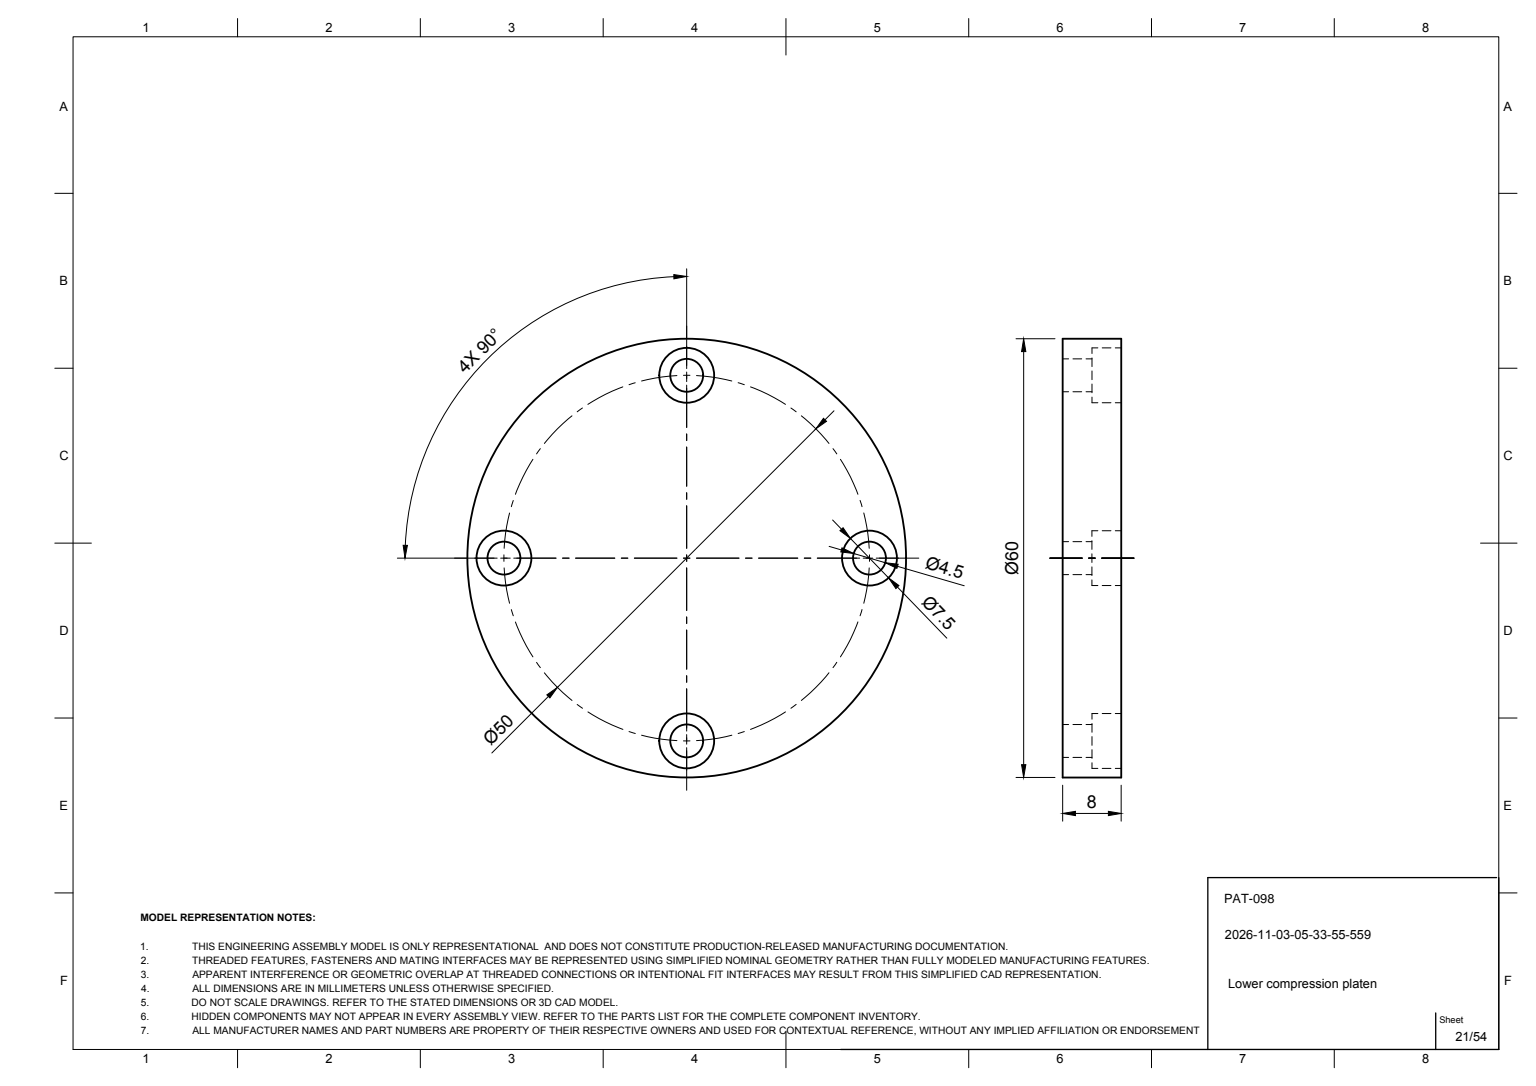
ISO-10303-21;
HEADER;
/* Generated by software containing ST-Developer
 * from STEP Tools, Inc. (www.steptools.com) 
 */

FILE_DESCRIPTION(
/* description */ ('Spring compression tester'),
/* implementation_level */ '2;1');

FILE_NAME(
/* name */ 'Lower compression platen.step',
/* time_stamp */ '2026-10-28T03:24:11-07:00',
/* author */ (''),
/* organization */ (''),
/* preprocessor_version */ 'ST-DEVELOPER v20.2',
/* originating_system */ 'Autodesk Translation Framework v15.17.0.0',
/* authorisation */ '');

FILE_SCHEMA (('AUTOMOTIVE_DESIGN { 1 0 10303 214 3 1 1 }'));
ENDSEC;

DATA;
#10=MECHANICAL_DESIGN_GEOMETRIC_PRESENTATION_REPRESENTATION('',(#1122),#43521);
#1002=SHAPE_REPRESENTATION_RELATIONSHIP('SRR','None',#43814,#1062);
#1062=ADVANCED_BREP_SHAPE_REPRESENTATION('',(#1197),#43474);
#1122=STYLED_ITEM('',(#44195),#1197);
#1197=MANIFOLD_SOLID_BREP('Body1',#18559);
#1398=FACE_BOUND('',#3604,.T.);
#1399=FACE_BOUND('',#3607,.T.);
#1400=FACE_BOUND('',#3610,.T.);
#1401=FACE_BOUND('',#3613,.T.);
#1402=FACE_BOUND('',#3620,.T.);
#1403=FACE_BOUND('',#3621,.T.);
#1404=FACE_BOUND('',#3622,.T.);
#1405=FACE_BOUND('',#3623,.T.);
#1406=FACE_BOUND('',#3625,.T.);
#1407=FACE_BOUND('',#3626,.T.);
#1408=FACE_BOUND('',#3627,.T.);
#1409=FACE_BOUND('',#3628,.T.);
#1722=PLANE('',#19752);
#1723=PLANE('',#19757);
#1724=PLANE('',#19762);
#1725=PLANE('',#19767);
#1726=PLANE('',#19780);
#1727=PLANE('',#19781);
#2404=FACE_OUTER_BOUND('',#3602,.T.);
#2405=FACE_OUTER_BOUND('',#3603,.T.);
#2406=FACE_OUTER_BOUND('',#3605,.T.);
#2407=FACE_OUTER_BOUND('',#3606,.T.);
#2408=FACE_OUTER_BOUND('',#3608,.T.);
#2409=FACE_OUTER_BOUND('',#3609,.T.);
#2410=FACE_OUTER_BOUND('',#3611,.T.);
#2411=FACE_OUTER_BOUND('',#3612,.T.);
#2412=FACE_OUTER_BOUND('',#3614,.T.);
#2413=FACE_OUTER_BOUND('',#3615,.T.);
#2414=FACE_OUTER_BOUND('',#3616,.T.);
#2415=FACE_OUTER_BOUND('',#3617,.T.);
#2416=FACE_OUTER_BOUND('',#3618,.T.);
#2417=FACE_OUTER_BOUND('',#3619,.T.);
#2418=FACE_OUTER_BOUND('',#3624,.T.);
#3602=EDGE_LOOP('',(#13231,#13232,#13233,#13234));
#3603=EDGE_LOOP('',(#13235));
#3604=EDGE_LOOP('',(#13236));
#3605=EDGE_LOOP('',(#13237,#13238,#13239,#13240));
#3606=EDGE_LOOP('',(#13241));
#3607=EDGE_LOOP('',(#13242));
#3608=EDGE_LOOP('',(#13243,#13244,#13245,#13246));
#3609=EDGE_LOOP('',(#13247));
#3610=EDGE_LOOP('',(#13248));
#3611=EDGE_LOOP('',(#13249,#13250,#13251,#13252));
#3612=EDGE_LOOP('',(#13253));
#3613=EDGE_LOOP('',(#13254));
#3614=EDGE_LOOP('',(#13255,#13256,#13257,#13258));
#3615=EDGE_LOOP('',(#13259,#13260,#13261,#13262));
#3616=EDGE_LOOP('',(#13263,#13264,#13265,#13266));
#3617=EDGE_LOOP('',(#13267,#13268,#13269,#13270));
#3618=EDGE_LOOP('',(#13271,#13272,#13273,#13274));
#3619=EDGE_LOOP('',(#13275));
#3620=EDGE_LOOP('',(#13276));
#3621=EDGE_LOOP('',(#13277));
#3622=EDGE_LOOP('',(#13278));
#3623=EDGE_LOOP('',(#13279));
#3624=EDGE_LOOP('',(#13280));
#3625=EDGE_LOOP('',(#13281));
#3626=EDGE_LOOP('',(#13282));
#3627=EDGE_LOOP('',(#13283));
#3628=EDGE_LOOP('',(#13284));
#4903=LINE('',#27556,#6335);
#4904=LINE('',#27565,#6336);
#4905=LINE('',#27574,#6337);
#4906=LINE('',#27583,#6338);
#4907=LINE('',#27591,#6339);
#4908=LINE('',#27595,#6340);
#4909=LINE('',#27599,#6341);
#4910=LINE('',#27603,#6342);
#4911=LINE('',#27608,#6343);
#6335=VECTOR('',#22427,0.375);
#6336=VECTOR('',#22438,0.375);
#6337=VECTOR('',#22449,0.375);
#6338=VECTOR('',#22460,0.375);
#6339=VECTOR('',#22471,0.225);
#6340=VECTOR('',#22476,0.225);
#6341=VECTOR('',#22481,0.225);
#6342=VECTOR('',#22486,0.225);
#6343=VECTOR('',#22491,3.);
#7680=CIRCLE('',#19750,0.375);
#7681=CIRCLE('',#19751,0.375);
#7682=CIRCLE('',#19753,0.225);
#7683=CIRCLE('',#19755,0.375);
#7684=CIRCLE('',#19756,0.375);
#7685=CIRCLE('',#19758,0.225);
#7686=CIRCLE('',#19760,0.375);
#7687=CIRCLE('',#19761,0.375);
#7688=CIRCLE('',#19763,0.225);
#7689=CIRCLE('',#19765,0.375);
#7690=CIRCLE('',#19766,0.375);
#7691=CIRCLE('',#19768,0.225);
#7692=CIRCLE('',#19770,0.225);
#7693=CIRCLE('',#19772,0.225);
#7694=CIRCLE('',#19774,0.225);
#7695=CIRCLE('',#19776,0.225);
#7696=CIRCLE('',#19778,3.);
#7697=CIRCLE('',#19779,3.);
#8474=VERTEX_POINT('',#27553);
#8475=VERTEX_POINT('',#27555);
#8476=VERTEX_POINT('',#27559);
#8477=VERTEX_POINT('',#27562);
#8478=VERTEX_POINT('',#27564);
#8479=VERTEX_POINT('',#27568);
#8480=VERTEX_POINT('',#27571);
#8481=VERTEX_POINT('',#27573);
#8482=VERTEX_POINT('',#27577);
#8483=VERTEX_POINT('',#27580);
#8484=VERTEX_POINT('',#27582);
#8485=VERTEX_POINT('',#27586);
#8486=VERTEX_POINT('',#27589);
#8487=VERTEX_POINT('',#27593);
#8488=VERTEX_POINT('',#27597);
#8489=VERTEX_POINT('',#27601);
#8490=VERTEX_POINT('',#27605);
#8491=VERTEX_POINT('',#27607);
#10280=EDGE_CURVE('',#8474,#8474,#7680,.T.);
#10281=EDGE_CURVE('',#8474,#8475,#4903,.T.);
#10282=EDGE_CURVE('',#8475,#8475,#7681,.T.);
#10283=EDGE_CURVE('',#8476,#8476,#7682,.T.);
#10284=EDGE_CURVE('',#8477,#8477,#7683,.T.);
#10285=EDGE_CURVE('',#8477,#8478,#4904,.T.);
#10286=EDGE_CURVE('',#8478,#8478,#7684,.T.);
#10287=EDGE_CURVE('',#8479,#8479,#7685,.T.);
#10288=EDGE_CURVE('',#8480,#8480,#7686,.T.);
#10289=EDGE_CURVE('',#8480,#8481,#4905,.T.);
#10290=EDGE_CURVE('',#8481,#8481,#7687,.T.);
#10291=EDGE_CURVE('',#8482,#8482,#7688,.T.);
#10292=EDGE_CURVE('',#8483,#8483,#7689,.T.);
#10293=EDGE_CURVE('',#8483,#8484,#4906,.T.);
#10294=EDGE_CURVE('',#8484,#8484,#7690,.T.);
#10295=EDGE_CURVE('',#8485,#8485,#7691,.T.);
#10296=EDGE_CURVE('',#8486,#8486,#7692,.T.);
#10297=EDGE_CURVE('',#8486,#8476,#4907,.T.);
#10298=EDGE_CURVE('',#8487,#8487,#7693,.T.);
#10299=EDGE_CURVE('',#8487,#8479,#4908,.T.);
#10300=EDGE_CURVE('',#8488,#8488,#7694,.T.);
#10301=EDGE_CURVE('',#8488,#8482,#4909,.T.);
#10302=EDGE_CURVE('',#8489,#8489,#7695,.T.);
#10303=EDGE_CURVE('',#8489,#8485,#4910,.T.);
#10304=EDGE_CURVE('',#8490,#8490,#7696,.T.);
#10305=EDGE_CURVE('',#8490,#8491,#4911,.T.);
#10306=EDGE_CURVE('',#8491,#8491,#7697,.T.);
#13231=ORIENTED_EDGE('',*,*,#10280,.F.);
#13232=ORIENTED_EDGE('',*,*,#10281,.T.);
#13233=ORIENTED_EDGE('',*,*,#10282,.F.);
#13234=ORIENTED_EDGE('',*,*,#10281,.F.);
#13235=ORIENTED_EDGE('',*,*,#10280,.T.);
#13236=ORIENTED_EDGE('',*,*,#10283,.F.);
#13237=ORIENTED_EDGE('',*,*,#10284,.F.);
#13238=ORIENTED_EDGE('',*,*,#10285,.T.);
#13239=ORIENTED_EDGE('',*,*,#10286,.F.);
#13240=ORIENTED_EDGE('',*,*,#10285,.F.);
#13241=ORIENTED_EDGE('',*,*,#10284,.T.);
#13242=ORIENTED_EDGE('',*,*,#10287,.F.);
#13243=ORIENTED_EDGE('',*,*,#10288,.F.);
#13244=ORIENTED_EDGE('',*,*,#10289,.T.);
#13245=ORIENTED_EDGE('',*,*,#10290,.F.);
#13246=ORIENTED_EDGE('',*,*,#10289,.F.);
#13247=ORIENTED_EDGE('',*,*,#10288,.T.);
#13248=ORIENTED_EDGE('',*,*,#10291,.F.);
#13249=ORIENTED_EDGE('',*,*,#10292,.F.);
#13250=ORIENTED_EDGE('',*,*,#10293,.T.);
#13251=ORIENTED_EDGE('',*,*,#10294,.F.);
#13252=ORIENTED_EDGE('',*,*,#10293,.F.);
#13253=ORIENTED_EDGE('',*,*,#10292,.T.);
#13254=ORIENTED_EDGE('',*,*,#10295,.F.);
#13255=ORIENTED_EDGE('',*,*,#10296,.F.);
#13256=ORIENTED_EDGE('',*,*,#10297,.T.);
#13257=ORIENTED_EDGE('',*,*,#10283,.T.);
#13258=ORIENTED_EDGE('',*,*,#10297,.F.);
#13259=ORIENTED_EDGE('',*,*,#10298,.F.);
#13260=ORIENTED_EDGE('',*,*,#10299,.T.);
#13261=ORIENTED_EDGE('',*,*,#10287,.T.);
#13262=ORIENTED_EDGE('',*,*,#10299,.F.);
#13263=ORIENTED_EDGE('',*,*,#10300,.F.);
#13264=ORIENTED_EDGE('',*,*,#10301,.T.);
#13265=ORIENTED_EDGE('',*,*,#10291,.T.);
#13266=ORIENTED_EDGE('',*,*,#10301,.F.);
#13267=ORIENTED_EDGE('',*,*,#10302,.F.);
#13268=ORIENTED_EDGE('',*,*,#10303,.T.);
#13269=ORIENTED_EDGE('',*,*,#10295,.T.);
#13270=ORIENTED_EDGE('',*,*,#10303,.F.);
#13271=ORIENTED_EDGE('',*,*,#10304,.F.);
#13272=ORIENTED_EDGE('',*,*,#10305,.T.);
#13273=ORIENTED_EDGE('',*,*,#10306,.T.);
#13274=ORIENTED_EDGE('',*,*,#10305,.F.);
#13275=ORIENTED_EDGE('',*,*,#10304,.T.);
#13276=ORIENTED_EDGE('',*,*,#10294,.T.);
#13277=ORIENTED_EDGE('',*,*,#10290,.T.);
#13278=ORIENTED_EDGE('',*,*,#10286,.T.);
#13279=ORIENTED_EDGE('',*,*,#10282,.T.);
#13280=ORIENTED_EDGE('',*,*,#10306,.F.);
#13281=ORIENTED_EDGE('',*,*,#10296,.T.);
#13282=ORIENTED_EDGE('',*,*,#10298,.T.);
#13283=ORIENTED_EDGE('',*,*,#10300,.T.);
#13284=ORIENTED_EDGE('',*,*,#10302,.T.);
#17206=CYLINDRICAL_SURFACE('',#19749,0.375);
#17207=CYLINDRICAL_SURFACE('',#19754,0.375);
#17208=CYLINDRICAL_SURFACE('',#19759,0.375);
#17209=CYLINDRICAL_SURFACE('',#19764,0.375);
#17210=CYLINDRICAL_SURFACE('',#19769,0.225);
#17211=CYLINDRICAL_SURFACE('',#19771,0.225);
#17212=CYLINDRICAL_SURFACE('',#19773,0.225);
#17213=CYLINDRICAL_SURFACE('',#19775,0.225);
#17214=CYLINDRICAL_SURFACE('',#19777,3.);
#17728=ADVANCED_FACE('',(#2404),#17206,.F.);
#17729=ADVANCED_FACE('',(#2405,#1398),#1722,.T.);
#17730=ADVANCED_FACE('',(#2406),#17207,.F.);
#17731=ADVANCED_FACE('',(#2407,#1399),#1723,.T.);
#17732=ADVANCED_FACE('',(#2408),#17208,.F.);
#17733=ADVANCED_FACE('',(#2409,#1400),#1724,.T.);
#17734=ADVANCED_FACE('',(#2410),#17209,.F.);
#17735=ADVANCED_FACE('',(#2411,#1401),#1725,.T.);
#17736=ADVANCED_FACE('',(#2412),#17210,.F.);
#17737=ADVANCED_FACE('',(#2413),#17211,.F.);
#17738=ADVANCED_FACE('',(#2414),#17212,.F.);
#17739=ADVANCED_FACE('',(#2415),#17213,.F.);
#17740=ADVANCED_FACE('',(#2416),#17214,.T.);
#17741=ADVANCED_FACE('',(#2417,#1402,#1403,#1404,#1405),#1726,.T.);
#17742=ADVANCED_FACE('',(#2418,#1406,#1407,#1408,#1409),#1727,.F.);
#18559=CLOSED_SHELL('',(#17728,#17729,#17730,#17731,#17732,#17733,#17734,
#17735,#17736,#17737,#17738,#17739,#17740,#17741,#17742));
#19748=AXIS2_PLACEMENT_3D('',#27551,#22421,#22422);
#19749=AXIS2_PLACEMENT_3D('',#27552,#22423,#22424);
#19750=AXIS2_PLACEMENT_3D('',#27554,#22425,#22426);
#19751=AXIS2_PLACEMENT_3D('',#27557,#22428,#22429);
#19752=AXIS2_PLACEMENT_3D('',#27558,#22430,#22431);
#19753=AXIS2_PLACEMENT_3D('',#27560,#22432,#22433);
#19754=AXIS2_PLACEMENT_3D('',#27561,#22434,#22435);
#19755=AXIS2_PLACEMENT_3D('',#27563,#22436,#22437);
#19756=AXIS2_PLACEMENT_3D('',#27566,#22439,#22440);
#19757=AXIS2_PLACEMENT_3D('',#27567,#22441,#22442);
#19758=AXIS2_PLACEMENT_3D('',#27569,#22443,#22444);
#19759=AXIS2_PLACEMENT_3D('',#27570,#22445,#22446);
#19760=AXIS2_PLACEMENT_3D('',#27572,#22447,#22448);
#19761=AXIS2_PLACEMENT_3D('',#27575,#22450,#22451);
#19762=AXIS2_PLACEMENT_3D('',#27576,#22452,#22453);
#19763=AXIS2_PLACEMENT_3D('',#27578,#22454,#22455);
#19764=AXIS2_PLACEMENT_3D('',#27579,#22456,#22457);
#19765=AXIS2_PLACEMENT_3D('',#27581,#22458,#22459);
#19766=AXIS2_PLACEMENT_3D('',#27584,#22461,#22462);
#19767=AXIS2_PLACEMENT_3D('',#27585,#22463,#22464);
#19768=AXIS2_PLACEMENT_3D('',#27587,#22465,#22466);
#19769=AXIS2_PLACEMENT_3D('',#27588,#22467,#22468);
#19770=AXIS2_PLACEMENT_3D('',#27590,#22469,#22470);
#19771=AXIS2_PLACEMENT_3D('',#27592,#22472,#22473);
#19772=AXIS2_PLACEMENT_3D('',#27594,#22474,#22475);
#19773=AXIS2_PLACEMENT_3D('',#27596,#22477,#22478);
#19774=AXIS2_PLACEMENT_3D('',#27598,#22479,#22480);
#19775=AXIS2_PLACEMENT_3D('',#27600,#22482,#22483);
#19776=AXIS2_PLACEMENT_3D('',#27602,#22484,#22485);
#19777=AXIS2_PLACEMENT_3D('',#27604,#22487,#22488);
#19778=AXIS2_PLACEMENT_3D('',#27606,#22489,#22490);
#19779=AXIS2_PLACEMENT_3D('',#27609,#22492,#22493);
#19780=AXIS2_PLACEMENT_3D('',#27610,#22494,#22495);
#19781=AXIS2_PLACEMENT_3D('',#27611,#22496,#22497);
#22421=DIRECTION('axis',(0.,0.,1.));
#22422=DIRECTION('refdir',(1.,0.,0.));
#22423=DIRECTION('center_axis',(0.,0.,1.));
#22424=DIRECTION('ref_axis',(1.,0.,0.));
#22425=DIRECTION('center_axis',(0.,0.,1.));
#22426=DIRECTION('ref_axis',(1.,0.,0.));
#22427=DIRECTION('',(0.,0.,1.));
#22428=DIRECTION('center_axis',(0.,0.,-1.));
#22429=DIRECTION('ref_axis',(1.,0.,0.));
#22430=DIRECTION('center_axis',(0.,0.,1.));
#22431=DIRECTION('ref_axis',(1.,0.,0.));
#22432=DIRECTION('center_axis',(0.,0.,1.));
#22433=DIRECTION('ref_axis',(1.,0.,0.));
#22434=DIRECTION('center_axis',(0.,0.,1.));
#22435=DIRECTION('ref_axis',(1.,0.,0.));
#22436=DIRECTION('center_axis',(0.,0.,1.));
#22437=DIRECTION('ref_axis',(1.,0.,0.));
#22438=DIRECTION('',(0.,0.,1.));
#22439=DIRECTION('center_axis',(0.,0.,-1.));
#22440=DIRECTION('ref_axis',(1.,0.,0.));
#22441=DIRECTION('center_axis',(0.,0.,1.));
#22442=DIRECTION('ref_axis',(1.,0.,0.));
#22443=DIRECTION('center_axis',(0.,0.,1.));
#22444=DIRECTION('ref_axis',(1.,0.,0.));
#22445=DIRECTION('center_axis',(0.,0.,1.));
#22446=DIRECTION('ref_axis',(1.,0.,0.));
#22447=DIRECTION('center_axis',(0.,0.,1.));
#22448=DIRECTION('ref_axis',(1.,0.,0.));
#22449=DIRECTION('',(0.,0.,1.));
#22450=DIRECTION('center_axis',(0.,0.,-1.));
#22451=DIRECTION('ref_axis',(1.,0.,0.));
#22452=DIRECTION('center_axis',(0.,0.,1.));
#22453=DIRECTION('ref_axis',(1.,0.,0.));
#22454=DIRECTION('center_axis',(0.,0.,1.));
#22455=DIRECTION('ref_axis',(1.,0.,0.));
#22456=DIRECTION('center_axis',(0.,0.,1.));
#22457=DIRECTION('ref_axis',(1.,0.,0.));
#22458=DIRECTION('center_axis',(0.,0.,1.));
#22459=DIRECTION('ref_axis',(1.,0.,0.));
#22460=DIRECTION('',(0.,0.,1.));
#22461=DIRECTION('center_axis',(0.,0.,-1.));
#22462=DIRECTION('ref_axis',(1.,0.,0.));
#22463=DIRECTION('center_axis',(0.,0.,1.));
#22464=DIRECTION('ref_axis',(1.,0.,0.));
#22465=DIRECTION('center_axis',(0.,0.,1.));
#22466=DIRECTION('ref_axis',(1.,0.,0.));
#22467=DIRECTION('center_axis',(0.,0.,1.));
#22468=DIRECTION('ref_axis',(1.,0.,0.));
#22469=DIRECTION('center_axis',(0.,0.,1.));
#22470=DIRECTION('ref_axis',(1.,0.,0.));
#22471=DIRECTION('',(0.,0.,1.));
#22472=DIRECTION('center_axis',(0.,0.,1.));
#22473=DIRECTION('ref_axis',(1.,0.,0.));
#22474=DIRECTION('center_axis',(0.,0.,1.));
#22475=DIRECTION('ref_axis',(1.,0.,0.));
#22476=DIRECTION('',(0.,0.,1.));
#22477=DIRECTION('center_axis',(0.,0.,1.));
#22478=DIRECTION('ref_axis',(1.,0.,0.));
#22479=DIRECTION('center_axis',(0.,0.,1.));
#22480=DIRECTION('ref_axis',(1.,0.,0.));
#22481=DIRECTION('',(0.,0.,1.));
#22482=DIRECTION('center_axis',(0.,0.,1.));
#22483=DIRECTION('ref_axis',(1.,0.,0.));
#22484=DIRECTION('center_axis',(0.,0.,1.));
#22485=DIRECTION('ref_axis',(1.,0.,0.));
#22486=DIRECTION('',(0.,0.,1.));
#22487=DIRECTION('center_axis',(0.,0.,1.));
#22488=DIRECTION('ref_axis',(1.,0.,0.));
#22489=DIRECTION('center_axis',(0.,0.,1.));
#22490=DIRECTION('ref_axis',(1.,0.,0.));
#22491=DIRECTION('',(0.,0.,-1.));
#22492=DIRECTION('center_axis',(0.,0.,1.));
#22493=DIRECTION('ref_axis',(1.,0.,0.));
#22494=DIRECTION('center_axis',(0.,0.,1.));
#22495=DIRECTION('ref_axis',(1.,0.,0.));
#22496=DIRECTION('center_axis',(0.,0.,1.));
#22497=DIRECTION('ref_axis',(1.,0.,0.));
#27551=CARTESIAN_POINT('',(0.,0.,0.));
#27552=CARTESIAN_POINT('Origin',(-2.5,-1.5,0.4));
#27553=CARTESIAN_POINT('',(-2.875,-1.5,0.4));
#27554=CARTESIAN_POINT('Origin',(-2.5,-1.5,0.4));
#27555=CARTESIAN_POINT('',(-2.875,-1.5,0.8));
#27556=CARTESIAN_POINT('',(-2.875,-1.5,0.4));
#27557=CARTESIAN_POINT('Origin',(-2.5,-1.5,0.8));
#27558=CARTESIAN_POINT('Origin',(-2.5,-1.5,0.4));
#27559=CARTESIAN_POINT('',(-2.725,-1.5,0.4));
#27560=CARTESIAN_POINT('Origin',(-2.5,-1.5,0.4));
#27561=CARTESIAN_POINT('Origin',(1.53080849893419E-16,1.,0.4));
#27562=CARTESIAN_POINT('',(-0.375,1.,0.4));
#27563=CARTESIAN_POINT('Origin',(1.53080849893419E-16,1.,0.4));
#27564=CARTESIAN_POINT('',(-0.375,1.,0.8));
#27565=CARTESIAN_POINT('',(-0.375,1.,0.4));
#27566=CARTESIAN_POINT('Origin',(1.53080849893419E-16,1.,0.8));
#27567=CARTESIAN_POINT('Origin',(1.66533453693773E-16,1.,0.4));
#27568=CARTESIAN_POINT('',(-0.225,1.,0.4));
#27569=CARTESIAN_POINT('Origin',(1.53080849893419E-16,1.,0.4));
#27570=CARTESIAN_POINT('Origin',(2.5,-1.5,0.4));
#27571=CARTESIAN_POINT('',(2.125,-1.5,0.4));
#27572=CARTESIAN_POINT('Origin',(2.5,-1.5,0.4));
#27573=CARTESIAN_POINT('',(2.125,-1.5,0.8));
#27574=CARTESIAN_POINT('',(2.125,-1.5,0.4));
#27575=CARTESIAN_POINT('Origin',(2.5,-1.5,0.8));
#27576=CARTESIAN_POINT('Origin',(2.5,-1.5,0.4));
#27577=CARTESIAN_POINT('',(2.275,-1.5,0.4));
#27578=CARTESIAN_POINT('Origin',(2.5,-1.5,0.4));
#27579=CARTESIAN_POINT('Origin',(-4.59242549680257E-16,-4.,0.4));
#27580=CARTESIAN_POINT('',(-0.375,-4.,0.4));
#27581=CARTESIAN_POINT('Origin',(-4.59242549680257E-16,-4.,0.4));
#27582=CARTESIAN_POINT('',(-0.375,-4.,0.8));
#27583=CARTESIAN_POINT('',(-0.375,-4.,0.4));
#27584=CARTESIAN_POINT('Origin',(-4.59242549680257E-16,-4.,0.8));
#27585=CARTESIAN_POINT('Origin',(-4.44089209850063E-16,-4.,0.4));
#27586=CARTESIAN_POINT('',(-0.225,-4.,0.4));
#27587=CARTESIAN_POINT('Origin',(-4.59242549680257E-16,-4.,0.4));
#27588=CARTESIAN_POINT('Origin',(-2.5,-1.5,-0.1));
#27589=CARTESIAN_POINT('',(-2.725,-1.5,0.));
#27590=CARTESIAN_POINT('Origin',(-2.5,-1.5,0.));
#27591=CARTESIAN_POINT('',(-2.725,-1.5,-0.1));
#27592=CARTESIAN_POINT('Origin',(1.53080849893419E-16,1.,-0.1));
#27593=CARTESIAN_POINT('',(-0.225,1.,0.));
#27594=CARTESIAN_POINT('Origin',(1.53080849893419E-16,1.,0.));
#27595=CARTESIAN_POINT('',(-0.225,1.,-0.1));
#27596=CARTESIAN_POINT('Origin',(2.5,-1.5,-0.1));
#27597=CARTESIAN_POINT('',(2.275,-1.5,0.));
#27598=CARTESIAN_POINT('Origin',(2.5,-1.5,0.));
#27599=CARTESIAN_POINT('',(2.275,-1.5,-0.1));
#27600=CARTESIAN_POINT('Origin',(-4.59242549680257E-16,-4.,-0.1));
#27601=CARTESIAN_POINT('',(-0.225,-4.,0.));
#27602=CARTESIAN_POINT('Origin',(-4.59242549680257E-16,-4.,0.));
#27603=CARTESIAN_POINT('',(-0.225,-4.,-0.1));
#27604=CARTESIAN_POINT('Origin',(0.,-1.5,0.));
#27605=CARTESIAN_POINT('',(-3.,-1.5,0.8));
#27606=CARTESIAN_POINT('Origin',(0.,-1.5,0.8));
#27607=CARTESIAN_POINT('',(-3.,-1.5,0.));
#27608=CARTESIAN_POINT('',(-3.,-1.5,0.));
#27609=CARTESIAN_POINT('Origin',(0.,-1.5,0.));
#27610=CARTESIAN_POINT('Origin',(0.,-1.5,0.8));
#27611=CARTESIAN_POINT('Origin',(0.,-1.5,0.));
#43406=UNCERTAINTY_MEASURE_WITH_UNIT(LENGTH_MEASURE(0.001),#43522,
'DISTANCE_ACCURACY_VALUE',
'Maximum model space distance between geometric entities at asserted c
onnectivities');
#43453=UNCERTAINTY_MEASURE_WITH_UNIT(LENGTH_MEASURE(0.001),#43522,
'DISTANCE_ACCURACY_VALUE',
'Maximum model space distance between geometric entities at asserted c
onnectivities');
#43474=(
GEOMETRIC_REPRESENTATION_CONTEXT(3)
GLOBAL_UNCERTAINTY_ASSIGNED_CONTEXT((#43406))
GLOBAL_UNIT_ASSIGNED_CONTEXT((#43522,#43524,#43525))
REPRESENTATION_CONTEXT('','3D')
);
#43521=(
GEOMETRIC_REPRESENTATION_CONTEXT(3)
GLOBAL_UNCERTAINTY_ASSIGNED_CONTEXT((#43453))
GLOBAL_UNIT_ASSIGNED_CONTEXT((#43522,#43524,#43525))
REPRESENTATION_CONTEXT('','3D')
);
#43522=(
LENGTH_UNIT()
NAMED_UNIT(*)
SI_UNIT(.CENTI.,.METRE.)
);
#43524=(
NAMED_UNIT(*)
PLANE_ANGLE_UNIT()
SI_UNIT($,.RADIAN.)
);
#43525=(
NAMED_UNIT(*)
SI_UNIT($,.STERADIAN.)
SOLID_ANGLE_UNIT()
);
#43546=SHAPE_DEFINITION_REPRESENTATION(#43613,#43814);
#43613=PRODUCT_DEFINITION_SHAPE('',$,#43882);
#43814=SHAPE_REPRESENTATION('',(#19748),#43474);
#43861=PRODUCT_DEFINITION_CONTEXT('part definition',#44064,'design');
#43882=PRODUCT_DEFINITION('Lower compression platen',
'Lower compression platen',#43949,#43861);
#43949=PRODUCT_DEFINITION_FORMATION('',$,#44086);
#44064=APPLICATION_CONTEXT(
'Core Data for Automotive Mechanical Design Process');
#44065=PRODUCT_CONTEXT('part definition',#44064,'mechanical');
#44086=PRODUCT('Lower compression platen','Lower compression platen',
'Lower compression platen',(#44065));
#44189=COLOUR_RGB('Sky Blue',0.24,0.69,0.87);
#44190=FILL_AREA_STYLE_COLOUR('',#44189);
#44191=FILL_AREA_STYLE('',(#44190));
#44192=SURFACE_STYLE_FILL_AREA(#44191);
#44193=SURFACE_SIDE_STYLE('',(#44192));
#44194=SURFACE_STYLE_USAGE(.BOTH.,#44193);
#44195=PRESENTATION_STYLE_ASSIGNMENT((#44194));
ENDSEC;
END-ISO-10303-21;
